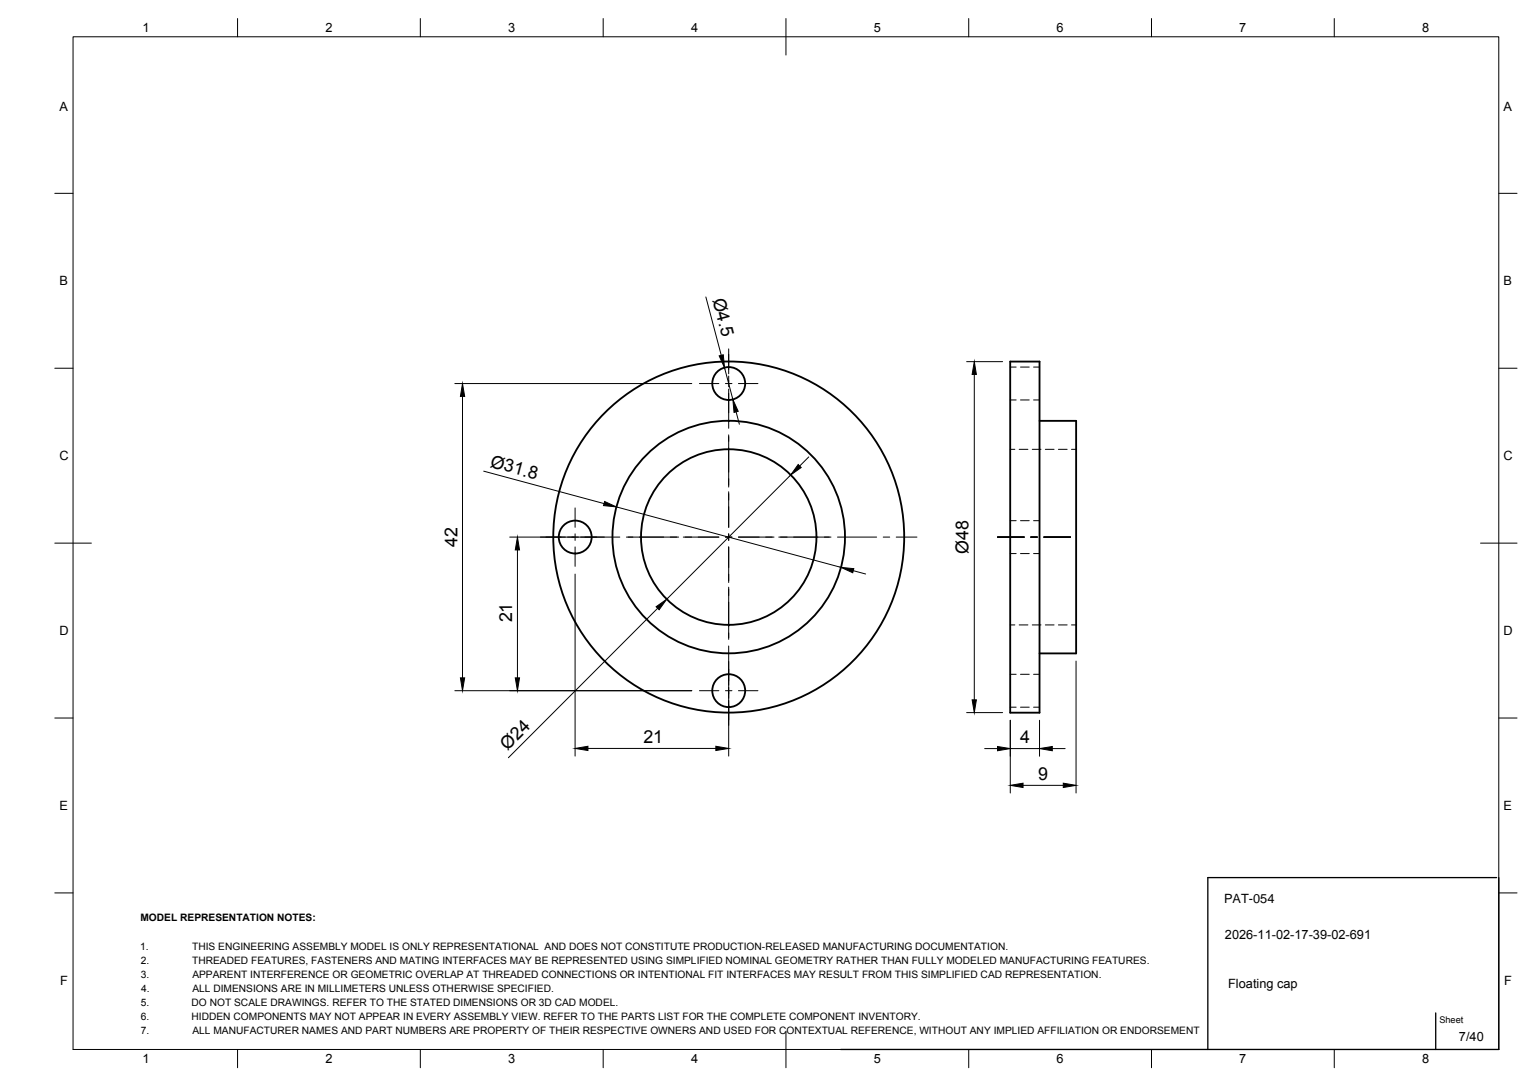
ISO-10303-21;
HEADER;
/* Generated by software containing ST-Developer
 * from STEP Tools, Inc. (www.steptools.com) 
 */

FILE_DESCRIPTION(
/* description */ ('PAT-054'),
/* implementation_level */ '2;1');

FILE_NAME(
/* name */ 'Floating cap.step',
/* time_stamp */ '2026-10-29T16:38:13-07:00',
/* author */ (''),
/* organization */ (''),
/* preprocessor_version */ 'ST-DEVELOPER v20.2',
/* originating_system */ 'Autodesk Translation Framework v15.17.0.0',
/* authorisation */ '');

FILE_SCHEMA (('AUTOMOTIVE_DESIGN { 1 0 10303 214 3 1 1 }'));
ENDSEC;

DATA;
#10=MECHANICAL_DESIGN_GEOMETRIC_PRESENTATION_REPRESENTATION('',(#902),#33981);
#814=SHAPE_REPRESENTATION_RELATIONSHIP('SRR','None',#34187,#858);
#858=ADVANCED_BREP_SHAPE_REPRESENTATION('',(#961),#33935);
#902=STYLED_ITEM('',(#34510),#961);
#961=MANIFOLD_SOLID_BREP('Body1',#13013);
#1075=FACE_BOUND('',#2426,.T.);
#1076=FACE_BOUND('',#2430,.T.);
#1077=FACE_BOUND('',#2431,.T.);
#1078=FACE_BOUND('',#2432,.T.);
#1079=FACE_BOUND('',#2433,.T.);
#1080=FACE_BOUND('',#2435,.T.);
#1081=FACE_BOUND('',#2436,.T.);
#1082=FACE_BOUND('',#2437,.T.);
#1083=FACE_BOUND('',#2438,.T.);
#1253=PLANE('',#13707);
#1254=PLANE('',#13714);
#1255=PLANE('',#13715);
#1635=FACE_OUTER_BOUND('',#2421,.T.);
#1636=FACE_OUTER_BOUND('',#2422,.T.);
#1637=FACE_OUTER_BOUND('',#2423,.T.);
#1638=FACE_OUTER_BOUND('',#2424,.T.);
#1639=FACE_OUTER_BOUND('',#2425,.T.);
#1640=FACE_OUTER_BOUND('',#2427,.T.);
#1641=FACE_OUTER_BOUND('',#2428,.T.);
#1642=FACE_OUTER_BOUND('',#2429,.T.);
#1643=FACE_OUTER_BOUND('',#2434,.T.);
#2421=EDGE_LOOP('',(#8771,#8772,#8773,#8774));
#2422=EDGE_LOOP('',(#8775,#8776,#8777,#8778));
#2423=EDGE_LOOP('',(#8779,#8780,#8781,#8782));
#2424=EDGE_LOOP('',(#8783,#8784,#8785,#8786));
#2425=EDGE_LOOP('',(#8787));
#2426=EDGE_LOOP('',(#8788));
#2427=EDGE_LOOP('',(#8789,#8790,#8791,#8792));
#2428=EDGE_LOOP('',(#8793,#8794,#8795,#8796));
#2429=EDGE_LOOP('',(#8797));
#2430=EDGE_LOOP('',(#8798));
#2431=EDGE_LOOP('',(#8799));
#2432=EDGE_LOOP('',(#8800));
#2433=EDGE_LOOP('',(#8801));
#2434=EDGE_LOOP('',(#8802));
#2435=EDGE_LOOP('',(#8803));
#2436=EDGE_LOOP('',(#8804));
#2437=EDGE_LOOP('',(#8805));
#2438=EDGE_LOOP('',(#8806));
#3308=LINE('',#18791,#4242);
#3309=LINE('',#18797,#4243);
#3310=LINE('',#18803,#4244);
#3311=LINE('',#18809,#4245);
#3312=LINE('',#18816,#4246);
#3313=LINE('',#18822,#4247);
#4242=VECTOR('',#15237,0.225);
#4243=VECTOR('',#15244,0.225);
#4244=VECTOR('',#15251,0.225);
#4245=VECTOR('',#15258,1.59);
#4246=VECTOR('',#15267,1.2);
#4247=VECTOR('',#15274,2.4);
#5175=CIRCLE('',#13696,0.225);
#5176=CIRCLE('',#13697,0.225);
#5177=CIRCLE('',#13699,0.225);
#5178=CIRCLE('',#13700,0.225);
#5179=CIRCLE('',#13702,0.225);
#5180=CIRCLE('',#13703,0.225);
#5181=CIRCLE('',#13705,1.59);
#5182=CIRCLE('',#13706,1.59);
#5183=CIRCLE('',#13708,1.2);
#5184=CIRCLE('',#13710,1.2);
#5185=CIRCLE('',#13712,2.4);
#5186=CIRCLE('',#13713,2.4);
#5664=VERTEX_POINT('',#18788);
#5665=VERTEX_POINT('',#18790);
#5666=VERTEX_POINT('',#18794);
#5667=VERTEX_POINT('',#18796);
#5668=VERTEX_POINT('',#18800);
#5669=VERTEX_POINT('',#18802);
#5670=VERTEX_POINT('',#18806);
#5671=VERTEX_POINT('',#18808);
#5672=VERTEX_POINT('',#18812);
#5673=VERTEX_POINT('',#18815);
#5674=VERTEX_POINT('',#18819);
#5675=VERTEX_POINT('',#18821);
#6885=EDGE_CURVE('',#5664,#5664,#5175,.T.);
#6886=EDGE_CURVE('',#5664,#5665,#3308,.T.);
#6887=EDGE_CURVE('',#5665,#5665,#5176,.T.);
#6888=EDGE_CURVE('',#5666,#5666,#5177,.T.);
#6889=EDGE_CURVE('',#5666,#5667,#3309,.T.);
#6890=EDGE_CURVE('',#5667,#5667,#5178,.T.);
#6891=EDGE_CURVE('',#5668,#5668,#5179,.T.);
#6892=EDGE_CURVE('',#5668,#5669,#3310,.T.);
#6893=EDGE_CURVE('',#5669,#5669,#5180,.T.);
#6894=EDGE_CURVE('',#5670,#5670,#5181,.T.);
#6895=EDGE_CURVE('',#5670,#5671,#3311,.T.);
#6896=EDGE_CURVE('',#5671,#5671,#5182,.T.);
#6897=EDGE_CURVE('',#5672,#5672,#5183,.T.);
#6898=EDGE_CURVE('',#5672,#5673,#3312,.T.);
#6899=EDGE_CURVE('',#5673,#5673,#5184,.T.);
#6900=EDGE_CURVE('',#5674,#5674,#5185,.T.);
#6901=EDGE_CURVE('',#5674,#5675,#3313,.T.);
#6902=EDGE_CURVE('',#5675,#5675,#5186,.T.);
#8771=ORIENTED_EDGE('',*,*,#6885,.F.);
#8772=ORIENTED_EDGE('',*,*,#6886,.T.);
#8773=ORIENTED_EDGE('',*,*,#6887,.F.);
#8774=ORIENTED_EDGE('',*,*,#6886,.F.);
#8775=ORIENTED_EDGE('',*,*,#6888,.F.);
#8776=ORIENTED_EDGE('',*,*,#6889,.T.);
#8777=ORIENTED_EDGE('',*,*,#6890,.F.);
#8778=ORIENTED_EDGE('',*,*,#6889,.F.);
#8779=ORIENTED_EDGE('',*,*,#6891,.F.);
#8780=ORIENTED_EDGE('',*,*,#6892,.T.);
#8781=ORIENTED_EDGE('',*,*,#6893,.F.);
#8782=ORIENTED_EDGE('',*,*,#6892,.F.);
#8783=ORIENTED_EDGE('',*,*,#6894,.F.);
#8784=ORIENTED_EDGE('',*,*,#6895,.T.);
#8785=ORIENTED_EDGE('',*,*,#6896,.F.);
#8786=ORIENTED_EDGE('',*,*,#6895,.F.);
#8787=ORIENTED_EDGE('',*,*,#6894,.T.);
#8788=ORIENTED_EDGE('',*,*,#6897,.T.);
#8789=ORIENTED_EDGE('',*,*,#6897,.F.);
#8790=ORIENTED_EDGE('',*,*,#6898,.T.);
#8791=ORIENTED_EDGE('',*,*,#6899,.T.);
#8792=ORIENTED_EDGE('',*,*,#6898,.F.);
#8793=ORIENTED_EDGE('',*,*,#6900,.F.);
#8794=ORIENTED_EDGE('',*,*,#6901,.T.);
#8795=ORIENTED_EDGE('',*,*,#6902,.T.);
#8796=ORIENTED_EDGE('',*,*,#6901,.F.);
#8797=ORIENTED_EDGE('',*,*,#6900,.T.);
#8798=ORIENTED_EDGE('',*,*,#6887,.T.);
#8799=ORIENTED_EDGE('',*,*,#6890,.T.);
#8800=ORIENTED_EDGE('',*,*,#6893,.T.);
#8801=ORIENTED_EDGE('',*,*,#6896,.T.);
#8802=ORIENTED_EDGE('',*,*,#6902,.F.);
#8803=ORIENTED_EDGE('',*,*,#6885,.T.);
#8804=ORIENTED_EDGE('',*,*,#6888,.T.);
#8805=ORIENTED_EDGE('',*,*,#6891,.T.);
#8806=ORIENTED_EDGE('',*,*,#6899,.F.);
#12014=CYLINDRICAL_SURFACE('',#13695,0.225);
#12015=CYLINDRICAL_SURFACE('',#13698,0.225);
#12016=CYLINDRICAL_SURFACE('',#13701,0.225);
#12017=CYLINDRICAL_SURFACE('',#13704,1.59);
#12018=CYLINDRICAL_SURFACE('',#13709,1.2);
#12019=CYLINDRICAL_SURFACE('',#13711,2.4);
#12347=ADVANCED_FACE('',(#1635),#12014,.F.);
#12348=ADVANCED_FACE('',(#1636),#12015,.F.);
#12349=ADVANCED_FACE('',(#1637),#12016,.F.);
#12350=ADVANCED_FACE('',(#1638),#12017,.T.);
#12351=ADVANCED_FACE('',(#1639,#1075),#1253,.T.);
#12352=ADVANCED_FACE('',(#1640),#12018,.F.);
#12353=ADVANCED_FACE('',(#1641),#12019,.T.);
#12354=ADVANCED_FACE('',(#1642,#1076,#1077,#1078,#1079),#1254,.T.);
#12355=ADVANCED_FACE('',(#1643,#1080,#1081,#1082,#1083),#1255,.F.);
#13013=CLOSED_SHELL('',(#12347,#12348,#12349,#12350,#12351,#12352,#12353,
#12354,#12355));
#13694=AXIS2_PLACEMENT_3D('',#18786,#15231,#15232);
#13695=AXIS2_PLACEMENT_3D('',#18787,#15233,#15234);
#13696=AXIS2_PLACEMENT_3D('',#18789,#15235,#15236);
#13697=AXIS2_PLACEMENT_3D('',#18792,#15238,#15239);
#13698=AXIS2_PLACEMENT_3D('',#18793,#15240,#15241);
#13699=AXIS2_PLACEMENT_3D('',#18795,#15242,#15243);
#13700=AXIS2_PLACEMENT_3D('',#18798,#15245,#15246);
#13701=AXIS2_PLACEMENT_3D('',#18799,#15247,#15248);
#13702=AXIS2_PLACEMENT_3D('',#18801,#15249,#15250);
#13703=AXIS2_PLACEMENT_3D('',#18804,#15252,#15253);
#13704=AXIS2_PLACEMENT_3D('',#18805,#15254,#15255);
#13705=AXIS2_PLACEMENT_3D('',#18807,#15256,#15257);
#13706=AXIS2_PLACEMENT_3D('',#18810,#15259,#15260);
#13707=AXIS2_PLACEMENT_3D('',#18811,#15261,#15262);
#13708=AXIS2_PLACEMENT_3D('',#18813,#15263,#15264);
#13709=AXIS2_PLACEMENT_3D('',#18814,#15265,#15266);
#13710=AXIS2_PLACEMENT_3D('',#18817,#15268,#15269);
#13711=AXIS2_PLACEMENT_3D('',#18818,#15270,#15271);
#13712=AXIS2_PLACEMENT_3D('',#18820,#15272,#15273);
#13713=AXIS2_PLACEMENT_3D('',#18823,#15275,#15276);
#13714=AXIS2_PLACEMENT_3D('',#18824,#15277,#15278);
#13715=AXIS2_PLACEMENT_3D('',#18825,#15279,#15280);
#15231=DIRECTION('axis',(0.,0.,1.));
#15232=DIRECTION('refdir',(1.,0.,0.));
#15233=DIRECTION('center_axis',(1.,0.,0.));
#15234=DIRECTION('ref_axis',(0.,0.,-1.));
#15235=DIRECTION('center_axis',(1.,0.,0.));
#15236=DIRECTION('ref_axis',(0.,0.,-1.));
#15237=DIRECTION('',(1.,0.,0.));
#15238=DIRECTION('center_axis',(-1.,0.,0.));
#15239=DIRECTION('ref_axis',(0.,0.,-1.));
#15240=DIRECTION('center_axis',(1.,0.,0.));
#15241=DIRECTION('ref_axis',(0.,0.,-1.));
#15242=DIRECTION('center_axis',(1.,0.,0.));
#15243=DIRECTION('ref_axis',(0.,0.,-1.));
#15244=DIRECTION('',(1.,0.,0.));
#15245=DIRECTION('center_axis',(-1.,0.,0.));
#15246=DIRECTION('ref_axis',(0.,0.,-1.));
#15247=DIRECTION('center_axis',(1.,0.,0.));
#15248=DIRECTION('ref_axis',(0.,0.,-1.));
#15249=DIRECTION('center_axis',(1.,0.,0.));
#15250=DIRECTION('ref_axis',(0.,0.,-1.));
#15251=DIRECTION('',(1.,0.,0.));
#15252=DIRECTION('center_axis',(-1.,0.,0.));
#15253=DIRECTION('ref_axis',(0.,0.,-1.));
#15254=DIRECTION('center_axis',(1.,0.,0.));
#15255=DIRECTION('ref_axis',(0.,0.,-1.));
#15256=DIRECTION('center_axis',(1.,0.,0.));
#15257=DIRECTION('ref_axis',(0.,0.,-1.));
#15258=DIRECTION('',(-1.,0.,0.));
#15259=DIRECTION('center_axis',(-1.,0.,0.));
#15260=DIRECTION('ref_axis',(0.,0.,-1.));
#15261=DIRECTION('center_axis',(1.,0.,0.));
#15262=DIRECTION('ref_axis',(0.,0.,-1.));
#15263=DIRECTION('center_axis',(-1.,0.,0.));
#15264=DIRECTION('ref_axis',(0.,0.,-1.));
#15265=DIRECTION('center_axis',(1.,0.,0.));
#15266=DIRECTION('ref_axis',(0.,0.,-1.));
#15267=DIRECTION('',(-1.,0.,0.));
#15268=DIRECTION('center_axis',(-1.,0.,0.));
#15269=DIRECTION('ref_axis',(0.,0.,-1.));
#15270=DIRECTION('center_axis',(1.,0.,0.));
#15271=DIRECTION('ref_axis',(0.,0.,-1.));
#15272=DIRECTION('center_axis',(1.,0.,0.));
#15273=DIRECTION('ref_axis',(0.,0.,-1.));
#15274=DIRECTION('',(-1.,0.,0.));
#15275=DIRECTION('center_axis',(1.,0.,0.));
#15276=DIRECTION('ref_axis',(0.,0.,-1.));
#15277=DIRECTION('center_axis',(1.,0.,0.));
#15278=DIRECTION('ref_axis',(0.,0.,-1.));
#15279=DIRECTION('center_axis',(1.,0.,0.));
#15280=DIRECTION('ref_axis',(0.,0.,-1.));
#18786=CARTESIAN_POINT('',(0.,0.,0.));
#18787=CARTESIAN_POINT('Origin',(1.5,-2.1,4.));
#18788=CARTESIAN_POINT('',(1.6,-2.1,4.225));
#18789=CARTESIAN_POINT('Origin',(1.6,-2.1,4.));
#18790=CARTESIAN_POINT('',(2.,-2.1,4.225));
#18791=CARTESIAN_POINT('',(1.5,-2.1,4.225));
#18792=CARTESIAN_POINT('Origin',(2.,-2.1,4.));
#18793=CARTESIAN_POINT('Origin',(1.5,2.1,4.));
#18794=CARTESIAN_POINT('',(1.6,2.1,4.225));
#18795=CARTESIAN_POINT('Origin',(1.6,2.1,4.));
#18796=CARTESIAN_POINT('',(2.,2.1,4.225));
#18797=CARTESIAN_POINT('',(1.5,2.1,4.225));
#18798=CARTESIAN_POINT('Origin',(2.,2.1,4.));
#18799=CARTESIAN_POINT('Origin',(1.5,0.,6.1));
#18800=CARTESIAN_POINT('',(1.6,-2.75545529808154E-17,6.325));
#18801=CARTESIAN_POINT('Origin',(1.6,0.,6.1));
#18802=CARTESIAN_POINT('',(2.,2.75545529808154E-17,6.325));
#18803=CARTESIAN_POINT('',(1.5,-2.75545529808154E-17,6.325));
#18804=CARTESIAN_POINT('Origin',(2.,0.,6.1));
#18805=CARTESIAN_POINT('Origin',(2.,0.,4.));
#18806=CARTESIAN_POINT('',(2.5,-1.94718841064429E-16,5.59));
#18807=CARTESIAN_POINT('Origin',(2.5,0.,4.));
#18808=CARTESIAN_POINT('',(2.,-1.94718841064429E-16,5.59));
#18809=CARTESIAN_POINT('',(2.,-1.94718841064429E-16,5.59));
#18810=CARTESIAN_POINT('Origin',(2.,0.,4.));
#18811=CARTESIAN_POINT('Origin',(2.5,0.,4.));
#18812=CARTESIAN_POINT('',(2.5,-1.46957615897682E-16,5.2));
#18813=CARTESIAN_POINT('Origin',(2.5,0.,4.));
#18814=CARTESIAN_POINT('Origin',(1.6,0.,4.));
#18815=CARTESIAN_POINT('',(1.6,-1.46957615897682E-16,5.2));
#18816=CARTESIAN_POINT('',(1.6,-1.46957615897682E-16,5.2));
#18817=CARTESIAN_POINT('Origin',(1.6,0.,4.));
#18818=CARTESIAN_POINT('Origin',(1.6,0.,4.));
#18819=CARTESIAN_POINT('',(2.,-2.93915231795365E-16,6.4));
#18820=CARTESIAN_POINT('Origin',(2.,0.,4.));
#18821=CARTESIAN_POINT('',(1.6,-2.93915231795365E-16,6.4));
#18822=CARTESIAN_POINT('',(1.6,-2.93915231795365E-16,6.4));
#18823=CARTESIAN_POINT('Origin',(1.6,0.,4.));
#18824=CARTESIAN_POINT('Origin',(2.,0.,4.));
#18825=CARTESIAN_POINT('Origin',(1.6,0.,4.));
#33883=UNCERTAINTY_MEASURE_WITH_UNIT(LENGTH_MEASURE(0.001),#33982,
'DISTANCE_ACCURACY_VALUE',
'Maximum model space distance between geometric entities at asserted c
onnectivities');
#33929=UNCERTAINTY_MEASURE_WITH_UNIT(LENGTH_MEASURE(0.001),#33982,
'DISTANCE_ACCURACY_VALUE',
'Maximum model space distance between geometric entities at asserted c
onnectivities');
#33935=(
GEOMETRIC_REPRESENTATION_CONTEXT(3)
GLOBAL_UNCERTAINTY_ASSIGNED_CONTEXT((#33883))
GLOBAL_UNIT_ASSIGNED_CONTEXT((#33982,#33984,#33985))
REPRESENTATION_CONTEXT('','3D')
);
#33981=(
GEOMETRIC_REPRESENTATION_CONTEXT(3)
GLOBAL_UNCERTAINTY_ASSIGNED_CONTEXT((#33929))
GLOBAL_UNIT_ASSIGNED_CONTEXT((#33982,#33984,#33985))
REPRESENTATION_CONTEXT('','3D')
);
#33982=(
LENGTH_UNIT()
NAMED_UNIT(*)
SI_UNIT(.CENTI.,.METRE.)
);
#33984=(
NAMED_UNIT(*)
PLANE_ANGLE_UNIT()
SI_UNIT($,.RADIAN.)
);
#33985=(
NAMED_UNIT(*)
SI_UNIT($,.STERADIAN.)
SOLID_ANGLE_UNIT()
);
#33991=SHAPE_DEFINITION_REPRESENTATION(#34042,#34187);
#34042=PRODUCT_DEFINITION_SHAPE('',$,#34239);
#34187=SHAPE_REPRESENTATION('',(#13694),#33935);
#34233=PRODUCT_DEFINITION_CONTEXT('part definition',#34388,'design');
#34239=PRODUCT_DEFINITION('Floating cap','Floating cap',#34290,#34233);
#34290=PRODUCT_DEFINITION_FORMATION('',$,#34395);
#34388=APPLICATION_CONTEXT(
'Core Data for Automotive Mechanical Design Process');
#34389=PRODUCT_CONTEXT('part definition',#34388,'mechanical');
#34395=PRODUCT('Floating cap','Floating cap','Floating cap',(#34389));
#34504=COLOUR_RGB('Sky Blue',0.24,0.69,0.87);
#34505=FILL_AREA_STYLE_COLOUR('',#34504);
#34506=FILL_AREA_STYLE('',(#34505));
#34507=SURFACE_STYLE_FILL_AREA(#34506);
#34508=SURFACE_SIDE_STYLE('',(#34507));
#34509=SURFACE_STYLE_USAGE(.BOTH.,#34508);
#34510=PRESENTATION_STYLE_ASSIGNMENT((#34509));
ENDSEC;
END-ISO-10303-21;
